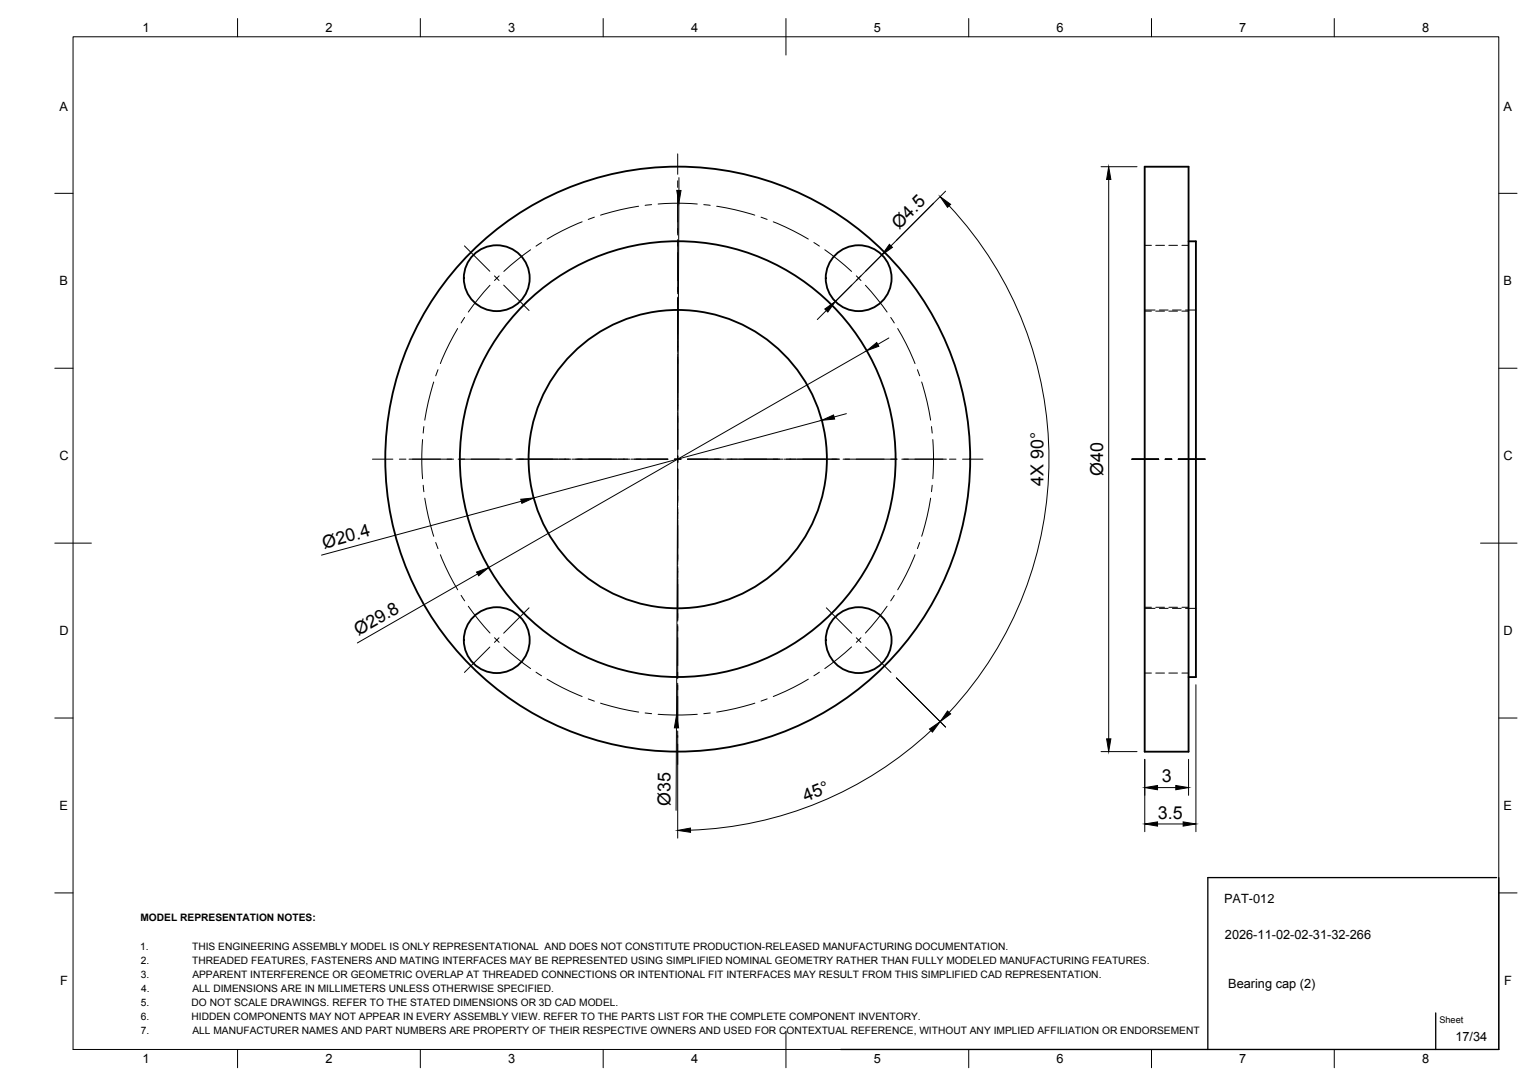
ISO-10303-21;
HEADER;
/* Generated by software containing ST-Developer
 * from STEP Tools, Inc. (www.steptools.com) 
 */

FILE_DESCRIPTION(
/* description */ ('Belt tensioner idler arm'),
/* implementation_level */ '2;1');

FILE_NAME(
/* name */ 'Bearing cap (2).step',
/* time_stamp */ '2026-10-28T03:22:15-07:00',
/* author */ (''),
/* organization */ (''),
/* preprocessor_version */ 'ST-DEVELOPER v20.2',
/* originating_system */ 'Autodesk Translation Framework v15.17.0.0',
/* authorisation */ '');

FILE_SCHEMA (('AUTOMOTIVE_DESIGN { 1 0 10303 214 3 1 1 }'));
ENDSEC;

DATA;
#10=MECHANICAL_DESIGN_GEOMETRIC_PRESENTATION_REPRESENTATION('',(#462),#12779);
#394=SHAPE_REPRESENTATION_RELATIONSHIP('SRR','None',#12941,#428);
#428=ADVANCED_BREP_SHAPE_REPRESENTATION('',(#502),#12758);
#462=STYLED_ITEM('',(#13184),#502);
#502=MANIFOLD_SOLID_BREP('Body1',#6198);
#604=FACE_BOUND('',#1442,.T.);
#605=FACE_BOUND('',#1446,.T.);
#606=FACE_BOUND('',#1447,.T.);
#607=FACE_BOUND('',#1448,.T.);
#608=FACE_BOUND('',#1449,.T.);
#609=FACE_BOUND('',#1450,.T.);
#610=FACE_BOUND('',#1452,.T.);
#611=FACE_BOUND('',#1453,.T.);
#612=FACE_BOUND('',#1454,.T.);
#613=FACE_BOUND('',#1455,.T.);
#614=FACE_BOUND('',#1456,.T.);
#750=PLANE('',#6916);
#751=PLANE('',#6923);
#752=PLANE('',#6924);
#992=FACE_OUTER_BOUND('',#1436,.T.);
#993=FACE_OUTER_BOUND('',#1437,.T.);
#994=FACE_OUTER_BOUND('',#1438,.T.);
#995=FACE_OUTER_BOUND('',#1439,.T.);
#996=FACE_OUTER_BOUND('',#1440,.T.);
#997=FACE_OUTER_BOUND('',#1441,.T.);
#998=FACE_OUTER_BOUND('',#1443,.T.);
#999=FACE_OUTER_BOUND('',#1444,.T.);
#1000=FACE_OUTER_BOUND('',#1445,.T.);
#1001=FACE_OUTER_BOUND('',#1451,.T.);
#1436=EDGE_LOOP('',(#4722,#4723,#4724,#4725));
#1437=EDGE_LOOP('',(#4726,#4727,#4728,#4729));
#1438=EDGE_LOOP('',(#4730,#4731,#4732,#4733));
#1439=EDGE_LOOP('',(#4734,#4735,#4736,#4737));
#1440=EDGE_LOOP('',(#4738,#4739,#4740,#4741));
#1441=EDGE_LOOP('',(#4742));
#1442=EDGE_LOOP('',(#4743));
#1443=EDGE_LOOP('',(#4744,#4745,#4746,#4747));
#1444=EDGE_LOOP('',(#4748,#4749,#4750,#4751));
#1445=EDGE_LOOP('',(#4752));
#1446=EDGE_LOOP('',(#4753));
#1447=EDGE_LOOP('',(#4754));
#1448=EDGE_LOOP('',(#4755));
#1449=EDGE_LOOP('',(#4756));
#1450=EDGE_LOOP('',(#4757));
#1451=EDGE_LOOP('',(#4758));
#1452=EDGE_LOOP('',(#4759));
#1453=EDGE_LOOP('',(#4760));
#1454=EDGE_LOOP('',(#4761));
#1455=EDGE_LOOP('',(#4762));
#1456=EDGE_LOOP('',(#4763));
#1875=LINE('',#10872,#2224);
#1876=LINE('',#10878,#2225);
#1877=LINE('',#10884,#2226);
#1878=LINE('',#10890,#2227);
#1879=LINE('',#10896,#2228);
#1880=LINE('',#10903,#2229);
#1881=LINE('',#10909,#2230);
#2224=VECTOR('',#8203,0.225);
#2225=VECTOR('',#8210,0.225);
#2226=VECTOR('',#8217,0.225);
#2227=VECTOR('',#8224,0.225);
#2228=VECTOR('',#8231,1.49);
#2229=VECTOR('',#8240,1.02);
#2230=VECTOR('',#8247,2.);
#2530=CIRCLE('',#6902,0.225);
#2531=CIRCLE('',#6903,0.225);
#2532=CIRCLE('',#6905,0.225);
#2533=CIRCLE('',#6906,0.225);
#2534=CIRCLE('',#6908,0.225);
#2535=CIRCLE('',#6909,0.225);
#2536=CIRCLE('',#6911,0.225);
#2537=CIRCLE('',#6912,0.225);
#2538=CIRCLE('',#6914,1.49);
#2539=CIRCLE('',#6915,1.49);
#2540=CIRCLE('',#6917,1.02);
#2541=CIRCLE('',#6919,1.02);
#2542=CIRCLE('',#6921,2.);
#2543=CIRCLE('',#6922,2.);
#2975=VERTEX_POINT('',#10869);
#2976=VERTEX_POINT('',#10871);
#2977=VERTEX_POINT('',#10875);
#2978=VERTEX_POINT('',#10877);
#2979=VERTEX_POINT('',#10881);
#2980=VERTEX_POINT('',#10883);
#2981=VERTEX_POINT('',#10887);
#2982=VERTEX_POINT('',#10889);
#2983=VERTEX_POINT('',#10893);
#2984=VERTEX_POINT('',#10895);
#2985=VERTEX_POINT('',#10899);
#2986=VERTEX_POINT('',#10902);
#2987=VERTEX_POINT('',#10906);
#2988=VERTEX_POINT('',#10908);
#3616=EDGE_CURVE('',#2975,#2975,#2530,.T.);
#3617=EDGE_CURVE('',#2975,#2976,#1875,.T.);
#3618=EDGE_CURVE('',#2976,#2976,#2531,.T.);
#3619=EDGE_CURVE('',#2977,#2977,#2532,.T.);
#3620=EDGE_CURVE('',#2977,#2978,#1876,.T.);
#3621=EDGE_CURVE('',#2978,#2978,#2533,.T.);
#3622=EDGE_CURVE('',#2979,#2979,#2534,.T.);
#3623=EDGE_CURVE('',#2979,#2980,#1877,.T.);
#3624=EDGE_CURVE('',#2980,#2980,#2535,.T.);
#3625=EDGE_CURVE('',#2981,#2981,#2536,.T.);
#3626=EDGE_CURVE('',#2981,#2982,#1878,.T.);
#3627=EDGE_CURVE('',#2982,#2982,#2537,.T.);
#3628=EDGE_CURVE('',#2983,#2983,#2538,.T.);
#3629=EDGE_CURVE('',#2983,#2984,#1879,.T.);
#3630=EDGE_CURVE('',#2984,#2984,#2539,.T.);
#3631=EDGE_CURVE('',#2985,#2985,#2540,.T.);
#3632=EDGE_CURVE('',#2985,#2986,#1880,.T.);
#3633=EDGE_CURVE('',#2986,#2986,#2541,.T.);
#3634=EDGE_CURVE('',#2987,#2987,#2542,.T.);
#3635=EDGE_CURVE('',#2987,#2988,#1881,.T.);
#3636=EDGE_CURVE('',#2988,#2988,#2543,.T.);
#4722=ORIENTED_EDGE('',*,*,#3616,.F.);
#4723=ORIENTED_EDGE('',*,*,#3617,.T.);
#4724=ORIENTED_EDGE('',*,*,#3618,.F.);
#4725=ORIENTED_EDGE('',*,*,#3617,.F.);
#4726=ORIENTED_EDGE('',*,*,#3619,.F.);
#4727=ORIENTED_EDGE('',*,*,#3620,.T.);
#4728=ORIENTED_EDGE('',*,*,#3621,.F.);
#4729=ORIENTED_EDGE('',*,*,#3620,.F.);
#4730=ORIENTED_EDGE('',*,*,#3622,.F.);
#4731=ORIENTED_EDGE('',*,*,#3623,.T.);
#4732=ORIENTED_EDGE('',*,*,#3624,.F.);
#4733=ORIENTED_EDGE('',*,*,#3623,.F.);
#4734=ORIENTED_EDGE('',*,*,#3625,.F.);
#4735=ORIENTED_EDGE('',*,*,#3626,.T.);
#4736=ORIENTED_EDGE('',*,*,#3627,.F.);
#4737=ORIENTED_EDGE('',*,*,#3626,.F.);
#4738=ORIENTED_EDGE('',*,*,#3628,.F.);
#4739=ORIENTED_EDGE('',*,*,#3629,.T.);
#4740=ORIENTED_EDGE('',*,*,#3630,.F.);
#4741=ORIENTED_EDGE('',*,*,#3629,.F.);
#4742=ORIENTED_EDGE('',*,*,#3628,.T.);
#4743=ORIENTED_EDGE('',*,*,#3631,.T.);
#4744=ORIENTED_EDGE('',*,*,#3631,.F.);
#4745=ORIENTED_EDGE('',*,*,#3632,.T.);
#4746=ORIENTED_EDGE('',*,*,#3633,.T.);
#4747=ORIENTED_EDGE('',*,*,#3632,.F.);
#4748=ORIENTED_EDGE('',*,*,#3634,.F.);
#4749=ORIENTED_EDGE('',*,*,#3635,.T.);
#4750=ORIENTED_EDGE('',*,*,#3636,.T.);
#4751=ORIENTED_EDGE('',*,*,#3635,.F.);
#4752=ORIENTED_EDGE('',*,*,#3634,.T.);
#4753=ORIENTED_EDGE('',*,*,#3630,.T.);
#4754=ORIENTED_EDGE('',*,*,#3627,.T.);
#4755=ORIENTED_EDGE('',*,*,#3624,.T.);
#4756=ORIENTED_EDGE('',*,*,#3621,.T.);
#4757=ORIENTED_EDGE('',*,*,#3618,.T.);
#4758=ORIENTED_EDGE('',*,*,#3636,.F.);
#4759=ORIENTED_EDGE('',*,*,#3633,.F.);
#4760=ORIENTED_EDGE('',*,*,#3625,.T.);
#4761=ORIENTED_EDGE('',*,*,#3622,.T.);
#4762=ORIENTED_EDGE('',*,*,#3619,.T.);
#4763=ORIENTED_EDGE('',*,*,#3616,.T.);
#5718=CYLINDRICAL_SURFACE('',#6901,0.225);
#5719=CYLINDRICAL_SURFACE('',#6904,0.225);
#5720=CYLINDRICAL_SURFACE('',#6907,0.225);
#5721=CYLINDRICAL_SURFACE('',#6910,0.225);
#5722=CYLINDRICAL_SURFACE('',#6913,1.49);
#5723=CYLINDRICAL_SURFACE('',#6918,1.02);
#5724=CYLINDRICAL_SURFACE('',#6920,2.);
#5969=ADVANCED_FACE('',(#992),#5718,.F.);
#5970=ADVANCED_FACE('',(#993),#5719,.F.);
#5971=ADVANCED_FACE('',(#994),#5720,.F.);
#5972=ADVANCED_FACE('',(#995),#5721,.F.);
#5973=ADVANCED_FACE('',(#996),#5722,.T.);
#5974=ADVANCED_FACE('',(#997,#604),#750,.T.);
#5975=ADVANCED_FACE('',(#998),#5723,.F.);
#5976=ADVANCED_FACE('',(#999),#5724,.T.);
#5977=ADVANCED_FACE('',(#1000,#605,#606,#607,#608,#609),#751,.T.);
#5978=ADVANCED_FACE('',(#1001,#610,#611,#612,#613,#614),#752,.F.);
#6198=CLOSED_SHELL('',(#5969,#5970,#5971,#5972,#5973,#5974,#5975,#5976,
#5977,#5978));
#6900=AXIS2_PLACEMENT_3D('',#10867,#8197,#8198);
#6901=AXIS2_PLACEMENT_3D('',#10868,#8199,#8200);
#6902=AXIS2_PLACEMENT_3D('',#10870,#8201,#8202);
#6903=AXIS2_PLACEMENT_3D('',#10873,#8204,#8205);
#6904=AXIS2_PLACEMENT_3D('',#10874,#8206,#8207);
#6905=AXIS2_PLACEMENT_3D('',#10876,#8208,#8209);
#6906=AXIS2_PLACEMENT_3D('',#10879,#8211,#8212);
#6907=AXIS2_PLACEMENT_3D('',#10880,#8213,#8214);
#6908=AXIS2_PLACEMENT_3D('',#10882,#8215,#8216);
#6909=AXIS2_PLACEMENT_3D('',#10885,#8218,#8219);
#6910=AXIS2_PLACEMENT_3D('',#10886,#8220,#8221);
#6911=AXIS2_PLACEMENT_3D('',#10888,#8222,#8223);
#6912=AXIS2_PLACEMENT_3D('',#10891,#8225,#8226);
#6913=AXIS2_PLACEMENT_3D('',#10892,#8227,#8228);
#6914=AXIS2_PLACEMENT_3D('',#10894,#8229,#8230);
#6915=AXIS2_PLACEMENT_3D('',#10897,#8232,#8233);
#6916=AXIS2_PLACEMENT_3D('',#10898,#8234,#8235);
#6917=AXIS2_PLACEMENT_3D('',#10900,#8236,#8237);
#6918=AXIS2_PLACEMENT_3D('',#10901,#8238,#8239);
#6919=AXIS2_PLACEMENT_3D('',#10904,#8241,#8242);
#6920=AXIS2_PLACEMENT_3D('',#10905,#8243,#8244);
#6921=AXIS2_PLACEMENT_3D('',#10907,#8245,#8246);
#6922=AXIS2_PLACEMENT_3D('',#10910,#8248,#8249);
#6923=AXIS2_PLACEMENT_3D('',#10911,#8250,#8251);
#6924=AXIS2_PLACEMENT_3D('',#10912,#8252,#8253);
#8197=DIRECTION('axis',(0.,0.,1.));
#8198=DIRECTION('refdir',(1.,0.,0.));
#8199=DIRECTION('center_axis',(0.,0.,1.));
#8200=DIRECTION('ref_axis',(1.,0.,0.));
#8201=DIRECTION('center_axis',(0.,0.,1.));
#8202=DIRECTION('ref_axis',(1.,0.,0.));
#8203=DIRECTION('',(0.,0.,1.));
#8204=DIRECTION('center_axis',(0.,0.,-1.));
#8205=DIRECTION('ref_axis',(1.,0.,0.));
#8206=DIRECTION('center_axis',(0.,0.,1.));
#8207=DIRECTION('ref_axis',(1.,0.,0.));
#8208=DIRECTION('center_axis',(0.,0.,1.));
#8209=DIRECTION('ref_axis',(1.,0.,0.));
#8210=DIRECTION('',(0.,0.,1.));
#8211=DIRECTION('center_axis',(0.,0.,-1.));
#8212=DIRECTION('ref_axis',(1.,0.,0.));
#8213=DIRECTION('center_axis',(0.,0.,1.));
#8214=DIRECTION('ref_axis',(1.,0.,0.));
#8215=DIRECTION('center_axis',(0.,0.,1.));
#8216=DIRECTION('ref_axis',(1.,0.,0.));
#8217=DIRECTION('',(0.,0.,1.));
#8218=DIRECTION('center_axis',(0.,0.,-1.));
#8219=DIRECTION('ref_axis',(1.,0.,0.));
#8220=DIRECTION('center_axis',(0.,0.,1.));
#8221=DIRECTION('ref_axis',(1.,0.,0.));
#8222=DIRECTION('center_axis',(0.,0.,1.));
#8223=DIRECTION('ref_axis',(1.,0.,0.));
#8224=DIRECTION('',(0.,0.,1.));
#8225=DIRECTION('center_axis',(0.,0.,-1.));
#8226=DIRECTION('ref_axis',(1.,0.,0.));
#8227=DIRECTION('center_axis',(0.,0.,1.));
#8228=DIRECTION('ref_axis',(1.,0.,0.));
#8229=DIRECTION('center_axis',(0.,0.,1.));
#8230=DIRECTION('ref_axis',(1.,0.,0.));
#8231=DIRECTION('',(0.,0.,-1.));
#8232=DIRECTION('center_axis',(0.,0.,-1.));
#8233=DIRECTION('ref_axis',(1.,0.,0.));
#8234=DIRECTION('center_axis',(0.,0.,1.));
#8235=DIRECTION('ref_axis',(1.,0.,0.));
#8236=DIRECTION('center_axis',(0.,0.,-1.));
#8237=DIRECTION('ref_axis',(1.,0.,0.));
#8238=DIRECTION('center_axis',(0.,0.,1.));
#8239=DIRECTION('ref_axis',(1.,0.,0.));
#8240=DIRECTION('',(0.,0.,-1.));
#8241=DIRECTION('center_axis',(0.,0.,-1.));
#8242=DIRECTION('ref_axis',(1.,0.,0.));
#8243=DIRECTION('center_axis',(0.,0.,1.));
#8244=DIRECTION('ref_axis',(1.,0.,0.));
#8245=DIRECTION('center_axis',(0.,0.,1.));
#8246=DIRECTION('ref_axis',(1.,0.,0.));
#8247=DIRECTION('',(0.,0.,-1.));
#8248=DIRECTION('center_axis',(0.,0.,1.));
#8249=DIRECTION('ref_axis',(1.,0.,0.));
#8250=DIRECTION('center_axis',(0.,0.,1.));
#8251=DIRECTION('ref_axis',(1.,0.,0.));
#8252=DIRECTION('center_axis',(0.,0.,1.));
#8253=DIRECTION('ref_axis',(1.,0.,0.));
#10867=CARTESIAN_POINT('',(0.,0.,0.));
#10868=CARTESIAN_POINT('Origin',(7.76256313292354,-1.23743686707646,4.6));
#10869=CARTESIAN_POINT('',(7.53756313292354,-1.23743686707646,4.7));
#10870=CARTESIAN_POINT('Origin',(7.76256313292354,-1.23743686707646,4.7));
#10871=CARTESIAN_POINT('',(7.53756313292354,-1.23743686707646,5.));
#10872=CARTESIAN_POINT('',(7.53756313292354,-1.23743686707646,4.6));
#10873=CARTESIAN_POINT('Origin',(7.76256313292354,-1.23743686707646,5.));
#10874=CARTESIAN_POINT('Origin',(7.76256313292354,1.23743686707646,4.6));
#10875=CARTESIAN_POINT('',(7.53756313292354,1.23743686707646,4.7));
#10876=CARTESIAN_POINT('Origin',(7.76256313292354,1.23743686707646,4.7));
#10877=CARTESIAN_POINT('',(7.53756313292354,1.23743686707646,5.));
#10878=CARTESIAN_POINT('',(7.53756313292354,1.23743686707646,4.6));
#10879=CARTESIAN_POINT('Origin',(7.76256313292354,1.23743686707646,5.));
#10880=CARTESIAN_POINT('Origin',(10.2374368670765,1.23743686707646,4.6));
#10881=CARTESIAN_POINT('',(10.0124368670765,1.23743686707646,4.7));
#10882=CARTESIAN_POINT('Origin',(10.2374368670765,1.23743686707646,4.7));
#10883=CARTESIAN_POINT('',(10.0124368670765,1.23743686707646,5.));
#10884=CARTESIAN_POINT('',(10.0124368670765,1.23743686707646,4.6));
#10885=CARTESIAN_POINT('Origin',(10.2374368670765,1.23743686707646,5.));
#10886=CARTESIAN_POINT('Origin',(10.2374368670765,-1.23743686707646,4.6));
#10887=CARTESIAN_POINT('',(10.0124368670765,-1.23743686707646,4.7));
#10888=CARTESIAN_POINT('Origin',(10.2374368670765,-1.23743686707646,4.7));
#10889=CARTESIAN_POINT('',(10.0124368670765,-1.23743686707646,5.));
#10890=CARTESIAN_POINT('',(10.0124368670765,-1.23743686707646,4.6));
#10891=CARTESIAN_POINT('Origin',(10.2374368670765,-1.23743686707646,5.));
#10892=CARTESIAN_POINT('Origin',(9.,0.,5.));
#10893=CARTESIAN_POINT('',(7.51,-1.82472373072956E-16,5.05));
#10894=CARTESIAN_POINT('Origin',(9.,0.,5.05));
#10895=CARTESIAN_POINT('',(7.51,-1.82472373072956E-16,5.));
#10896=CARTESIAN_POINT('',(7.51,-1.82472373072956E-16,5.));
#10897=CARTESIAN_POINT('Origin',(9.,0.,5.));
#10898=CARTESIAN_POINT('Origin',(9.,0.,5.05));
#10899=CARTESIAN_POINT('',(7.98,-1.2491397351303E-16,5.05));
#10900=CARTESIAN_POINT('Origin',(9.,0.,5.05));
#10901=CARTESIAN_POINT('Origin',(9.,0.,4.7));
#10902=CARTESIAN_POINT('',(7.98,-1.2491397351303E-16,4.7));
#10903=CARTESIAN_POINT('',(7.98,-1.2491397351303E-16,4.7));
#10904=CARTESIAN_POINT('Origin',(9.,0.,4.7));
#10905=CARTESIAN_POINT('Origin',(9.,0.,4.7));
#10906=CARTESIAN_POINT('',(7.,-2.44929359829471E-16,5.));
#10907=CARTESIAN_POINT('Origin',(9.,0.,5.));
#10908=CARTESIAN_POINT('',(7.,-2.44929359829471E-16,4.7));
#10909=CARTESIAN_POINT('',(7.,-2.44929359829471E-16,4.7));
#10910=CARTESIAN_POINT('Origin',(9.,0.,4.7));
#10911=CARTESIAN_POINT('Origin',(9.,0.,5.));
#10912=CARTESIAN_POINT('Origin',(9.,0.,4.7));
#12718=UNCERTAINTY_MEASURE_WITH_UNIT(LENGTH_MEASURE(0.001),#12780,
'DISTANCE_ACCURACY_VALUE',
'Maximum model space distance between geometric entities at asserted c
onnectivities');
#12739=UNCERTAINTY_MEASURE_WITH_UNIT(LENGTH_MEASURE(0.001),#12780,
'DISTANCE_ACCURACY_VALUE',
'Maximum model space distance between geometric entities at asserted c
onnectivities');
#12758=(
GEOMETRIC_REPRESENTATION_CONTEXT(3)
GLOBAL_UNCERTAINTY_ASSIGNED_CONTEXT((#12718))
GLOBAL_UNIT_ASSIGNED_CONTEXT((#12780,#12782,#12783))
REPRESENTATION_CONTEXT('','3D')
);
#12779=(
GEOMETRIC_REPRESENTATION_CONTEXT(3)
GLOBAL_UNCERTAINTY_ASSIGNED_CONTEXT((#12739))
GLOBAL_UNIT_ASSIGNED_CONTEXT((#12780,#12782,#12783))
REPRESENTATION_CONTEXT('','3D')
);
#12780=(
LENGTH_UNIT()
NAMED_UNIT(*)
SI_UNIT(.CENTI.,.METRE.)
);
#12782=(
NAMED_UNIT(*)
PLANE_ANGLE_UNIT()
SI_UNIT($,.RADIAN.)
);
#12783=(
NAMED_UNIT(*)
SI_UNIT($,.STERADIAN.)
SOLID_ANGLE_UNIT()
);
#12802=SHAPE_DEFINITION_REPRESENTATION(#12841,#12941);
#12841=PRODUCT_DEFINITION_SHAPE('',$,#12981);
#12941=SHAPE_REPRESENTATION('',(#6900),#12758);
#12962=PRODUCT_DEFINITION_CONTEXT('part definition',#13081,'design');
#12981=PRODUCT_DEFINITION('Bearing cap (2)','Bearing cap (2)',#13020,#12962);
#13020=PRODUCT_DEFINITION_FORMATION('',$,#13101);
#13081=APPLICATION_CONTEXT(
'Core Data for Automotive Mechanical Design Process');
#13082=PRODUCT_CONTEXT('part definition',#13081,'mechanical');
#13101=PRODUCT('Bearing cap (2)','Bearing cap (2)','Bearing cap (2)',(#13082));
#13178=COLOUR_RGB('Grey',0.48,0.52,0.57);
#13179=FILL_AREA_STYLE_COLOUR('',#13178);
#13180=FILL_AREA_STYLE('',(#13179));
#13181=SURFACE_STYLE_FILL_AREA(#13180);
#13182=SURFACE_SIDE_STYLE('',(#13181));
#13183=SURFACE_STYLE_USAGE(.BOTH.,#13182);
#13184=PRESENTATION_STYLE_ASSIGNMENT((#13183));
ENDSEC;
END-ISO-10303-21;
